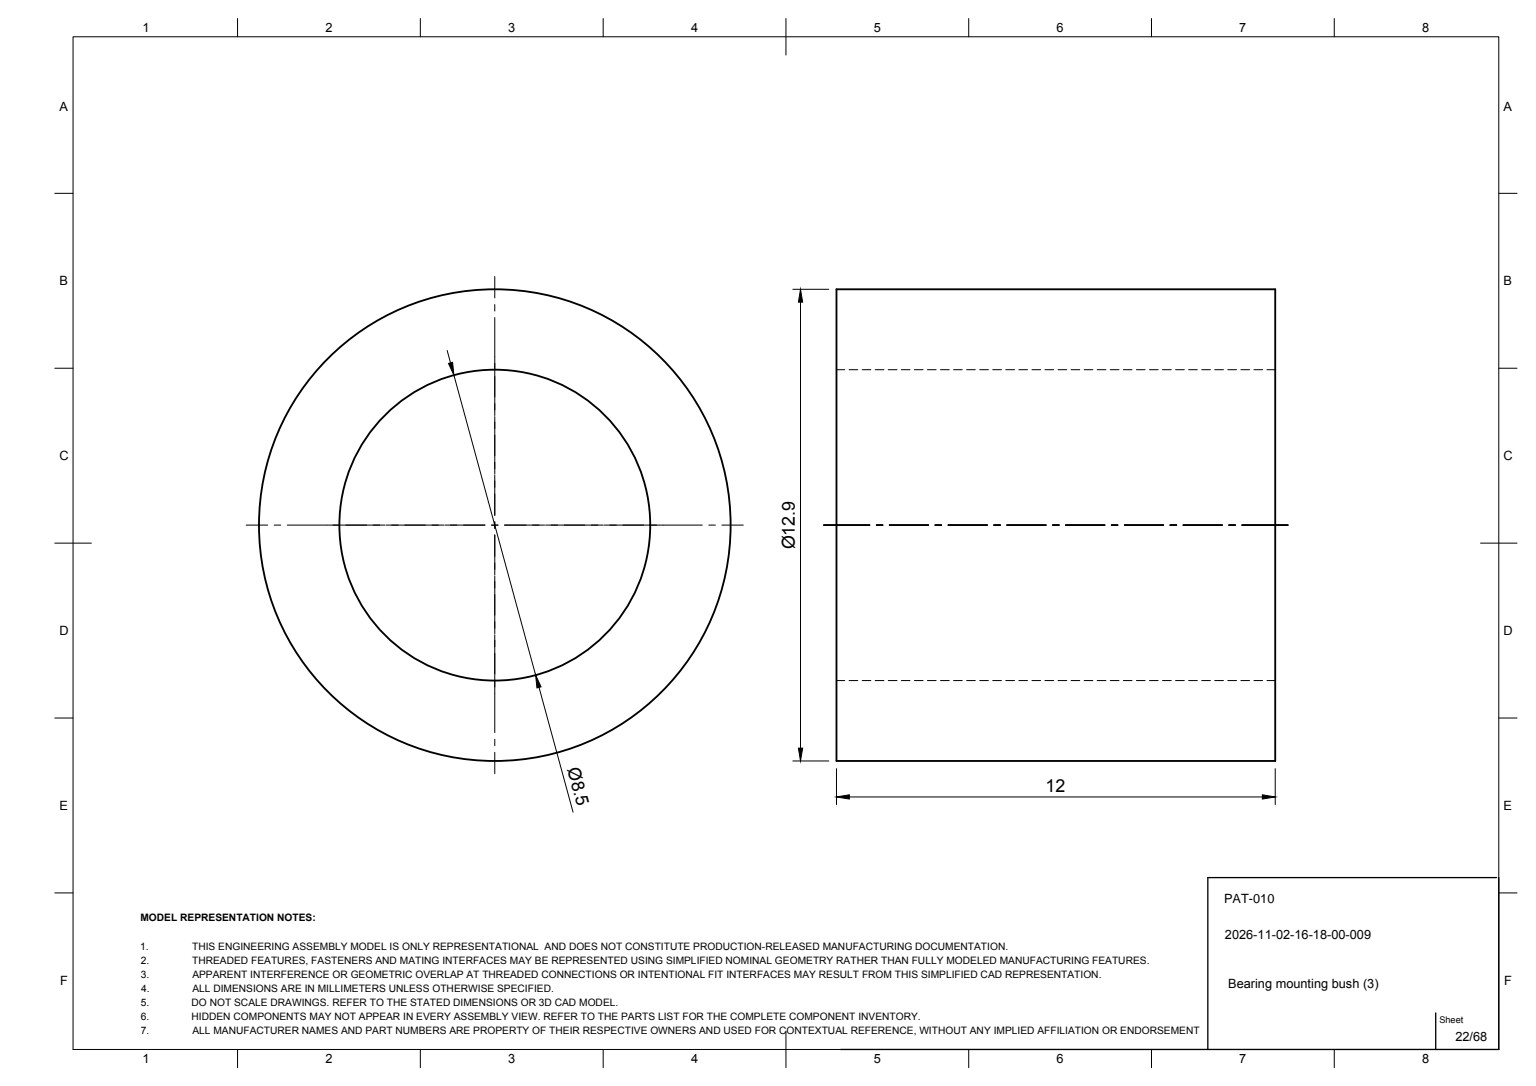
ISO-10303-21;
HEADER;
/* Generated by software containing ST-Developer
 * from STEP Tools, Inc. (www.steptools.com) 
 */

FILE_DESCRIPTION(
/* description */ ('Belt conveyor head drive unit'),
/* implementation_level */ '2;1');

FILE_NAME(
/* name */ 'Bearing mounting bush (3).step',
/* time_stamp */ '2026-10-28T03:26:19-07:00',
/* author */ (''),
/* organization */ (''),
/* preprocessor_version */ 'ST-DEVELOPER v20.2',
/* originating_system */ 'Autodesk Translation Framework v15.17.0.0',
/* authorisation */ '');

FILE_SCHEMA (('AUTOMOTIVE_DESIGN { 1 0 10303 214 3 1 1 }'));
ENDSEC;

DATA;
#10=MECHANICAL_DESIGN_GEOMETRIC_PRESENTATION_REPRESENTATION('',(#868),#27069);
#730=SHAPE_REPRESENTATION_RELATIONSHIP('SRR','None',#27374,#799);
#799=ADVANCED_BREP_SHAPE_REPRESENTATION('',(#953),#27016);
#868=STYLED_ITEM('',(#27797),#953);
#953=MANIFOLD_SOLID_BREP('Body1',#13733);
#1127=FACE_BOUND('',#2805,.T.);
#1128=FACE_BOUND('',#2807,.T.);
#1403=PLANE('',#15114);
#1404=PLANE('',#15115);
#1887=FACE_OUTER_BOUND('',#2802,.T.);
#1888=FACE_OUTER_BOUND('',#2803,.T.);
#1889=FACE_OUTER_BOUND('',#2804,.T.);
#1890=FACE_OUTER_BOUND('',#2806,.T.);
#2802=EDGE_LOOP('',(#10068,#10069,#10070,#10071));
#2803=EDGE_LOOP('',(#10072,#10073,#10074,#10075));
#2804=EDGE_LOOP('',(#10076));
#2805=EDGE_LOOP('',(#10077));
#2806=EDGE_LOOP('',(#10078));
#2807=EDGE_LOOP('',(#10079));
#3785=LINE('',#22177,#4577);
#3786=LINE('',#22183,#4578);
#4577=VECTOR('',#17817,0.425000000000001);
#4578=VECTOR('',#17824,0.645);
#5350=CIRCLE('',#15109,0.425000000000001);
#5351=CIRCLE('',#15110,0.425000000000001);
#5352=CIRCLE('',#15112,0.645);
#5353=CIRCLE('',#15113,0.645);
#6323=VERTEX_POINT('',#22174);
#6324=VERTEX_POINT('',#22176);
#6325=VERTEX_POINT('',#22180);
#6326=VERTEX_POINT('',#22182);
#7726=EDGE_CURVE('',#6323,#6323,#5350,.T.);
#7727=EDGE_CURVE('',#6323,#6324,#3785,.T.);
#7728=EDGE_CURVE('',#6324,#6324,#5351,.T.);
#7729=EDGE_CURVE('',#6325,#6325,#5352,.T.);
#7730=EDGE_CURVE('',#6325,#6326,#3786,.T.);
#7731=EDGE_CURVE('',#6326,#6326,#5353,.T.);
#10068=ORIENTED_EDGE('',*,*,#7726,.F.);
#10069=ORIENTED_EDGE('',*,*,#7727,.T.);
#10070=ORIENTED_EDGE('',*,*,#7728,.T.);
#10071=ORIENTED_EDGE('',*,*,#7727,.F.);
#10072=ORIENTED_EDGE('',*,*,#7729,.F.);
#10073=ORIENTED_EDGE('',*,*,#7730,.T.);
#10074=ORIENTED_EDGE('',*,*,#7731,.T.);
#10075=ORIENTED_EDGE('',*,*,#7730,.F.);
#10076=ORIENTED_EDGE('',*,*,#7729,.T.);
#10077=ORIENTED_EDGE('',*,*,#7726,.T.);
#10078=ORIENTED_EDGE('',*,*,#7731,.F.);
#10079=ORIENTED_EDGE('',*,*,#7728,.F.);
#12660=CYLINDRICAL_SURFACE('',#15108,0.425000000000001);
#12661=CYLINDRICAL_SURFACE('',#15111,0.645);
#13166=ADVANCED_FACE('',(#1887),#12660,.F.);
#13167=ADVANCED_FACE('',(#1888),#12661,.T.);
#13168=ADVANCED_FACE('',(#1889,#1127),#1403,.T.);
#13169=ADVANCED_FACE('',(#1890,#1128),#1404,.F.);
#13733=CLOSED_SHELL('',(#13166,#13167,#13168,#13169));
#15107=AXIS2_PLACEMENT_3D('',#22172,#17811,#17812);
#15108=AXIS2_PLACEMENT_3D('',#22173,#17813,#17814);
#15109=AXIS2_PLACEMENT_3D('',#22175,#17815,#17816);
#15110=AXIS2_PLACEMENT_3D('',#22178,#17818,#17819);
#15111=AXIS2_PLACEMENT_3D('',#22179,#17820,#17821);
#15112=AXIS2_PLACEMENT_3D('',#22181,#17822,#17823);
#15113=AXIS2_PLACEMENT_3D('',#22184,#17825,#17826);
#15114=AXIS2_PLACEMENT_3D('',#22185,#17827,#17828);
#15115=AXIS2_PLACEMENT_3D('',#22186,#17829,#17830);
#17811=DIRECTION('axis',(0.,0.,1.));
#17812=DIRECTION('refdir',(1.,0.,0.));
#17813=DIRECTION('center_axis',(0.,0.,1.));
#17814=DIRECTION('ref_axis',(1.,0.,0.));
#17815=DIRECTION('center_axis',(0.,0.,-1.));
#17816=DIRECTION('ref_axis',(1.,0.,0.));
#17817=DIRECTION('',(0.,0.,-1.));
#17818=DIRECTION('center_axis',(0.,0.,-1.));
#17819=DIRECTION('ref_axis',(1.,0.,0.));
#17820=DIRECTION('center_axis',(0.,0.,1.));
#17821=DIRECTION('ref_axis',(1.,0.,0.));
#17822=DIRECTION('center_axis',(0.,0.,1.));
#17823=DIRECTION('ref_axis',(1.,0.,0.));
#17824=DIRECTION('',(0.,0.,-1.));
#17825=DIRECTION('center_axis',(0.,0.,1.));
#17826=DIRECTION('ref_axis',(1.,0.,0.));
#17827=DIRECTION('center_axis',(0.,0.,1.));
#17828=DIRECTION('ref_axis',(1.,0.,0.));
#17829=DIRECTION('center_axis',(0.,0.,1.));
#17830=DIRECTION('ref_axis',(1.,0.,0.));
#22172=CARTESIAN_POINT('',(0.,0.,0.));
#22173=CARTESIAN_POINT('Origin',(11.7209100301812,40.,3.67));
#22174=CARTESIAN_POINT('',(11.2959100301812,40.,4.87));
#22175=CARTESIAN_POINT('Origin',(11.7209100301812,40.,4.87));
#22176=CARTESIAN_POINT('',(11.2959100301812,40.,3.67));
#22177=CARTESIAN_POINT('',(11.2959100301812,40.,3.67));
#22178=CARTESIAN_POINT('Origin',(11.7209100301812,40.,3.67));
#22179=CARTESIAN_POINT('Origin',(11.7209100301812,40.,3.67));
#22180=CARTESIAN_POINT('',(11.0759100301812,40.,4.87));
#22181=CARTESIAN_POINT('Origin',(11.7209100301812,40.,4.87));
#22182=CARTESIAN_POINT('',(11.0759100301812,40.,3.67));
#22183=CARTESIAN_POINT('',(11.0759100301812,40.,3.67));
#22184=CARTESIAN_POINT('Origin',(11.7209100301812,40.,3.67));
#22185=CARTESIAN_POINT('Origin',(11.7209100301812,40.,4.87));
#22186=CARTESIAN_POINT('Origin',(11.7209100301812,40.,3.67));
#26939=UNCERTAINTY_MEASURE_WITH_UNIT(LENGTH_MEASURE(0.001),#27070,
'DISTANCE_ACCURACY_VALUE',
'Maximum model space distance between geometric entities at asserted c
onnectivities');
#26992=UNCERTAINTY_MEASURE_WITH_UNIT(LENGTH_MEASURE(0.001),#27070,
'DISTANCE_ACCURACY_VALUE',
'Maximum model space distance between geometric entities at asserted c
onnectivities');
#27016=(
GEOMETRIC_REPRESENTATION_CONTEXT(3)
GLOBAL_UNCERTAINTY_ASSIGNED_CONTEXT((#26939))
GLOBAL_UNIT_ASSIGNED_CONTEXT((#27070,#27072,#27073))
REPRESENTATION_CONTEXT('','3D')
);
#27069=(
GEOMETRIC_REPRESENTATION_CONTEXT(3)
GLOBAL_UNCERTAINTY_ASSIGNED_CONTEXT((#26992))
GLOBAL_UNIT_ASSIGNED_CONTEXT((#27070,#27072,#27073))
REPRESENTATION_CONTEXT('','3D')
);
#27070=(
LENGTH_UNIT()
NAMED_UNIT(*)
SI_UNIT(.CENTI.,.METRE.)
);
#27072=(
NAMED_UNIT(*)
PLANE_ANGLE_UNIT()
SI_UNIT($,.RADIAN.)
);
#27073=(
NAMED_UNIT(*)
SI_UNIT($,.STERADIAN.)
SOLID_ANGLE_UNIT()
);
#27097=SHAPE_DEFINITION_REPRESENTATION(#27173,#27374);
#27173=PRODUCT_DEFINITION_SHAPE('',$,#27451);
#27374=SHAPE_REPRESENTATION('',(#15107),#27016);
#27427=PRODUCT_DEFINITION_CONTEXT('part definition',#27657,'design');
#27451=PRODUCT_DEFINITION('Bearing mounting bush (3)',
'Bearing mounting bush (3)',#27527,#27427);
#27527=PRODUCT_DEFINITION_FORMATION('',$,#27682);
#27657=APPLICATION_CONTEXT(
'Core Data for Automotive Mechanical Design Process');
#27658=PRODUCT_CONTEXT('part definition',#27657,'mechanical');
#27682=PRODUCT('Bearing mounting bush (3)','Bearing mounting bush (3)',
'Bearing mounting bush (3)',(#27658));
#27791=COLOUR_RGB('Grey',0.48,0.52,0.57);
#27792=FILL_AREA_STYLE_COLOUR('',#27791);
#27793=FILL_AREA_STYLE('',(#27792));
#27794=SURFACE_STYLE_FILL_AREA(#27793);
#27795=SURFACE_SIDE_STYLE('',(#27794));
#27796=SURFACE_STYLE_USAGE(.BOTH.,#27795);
#27797=PRESENTATION_STYLE_ASSIGNMENT((#27796));
ENDSEC;
END-ISO-10303-21;
